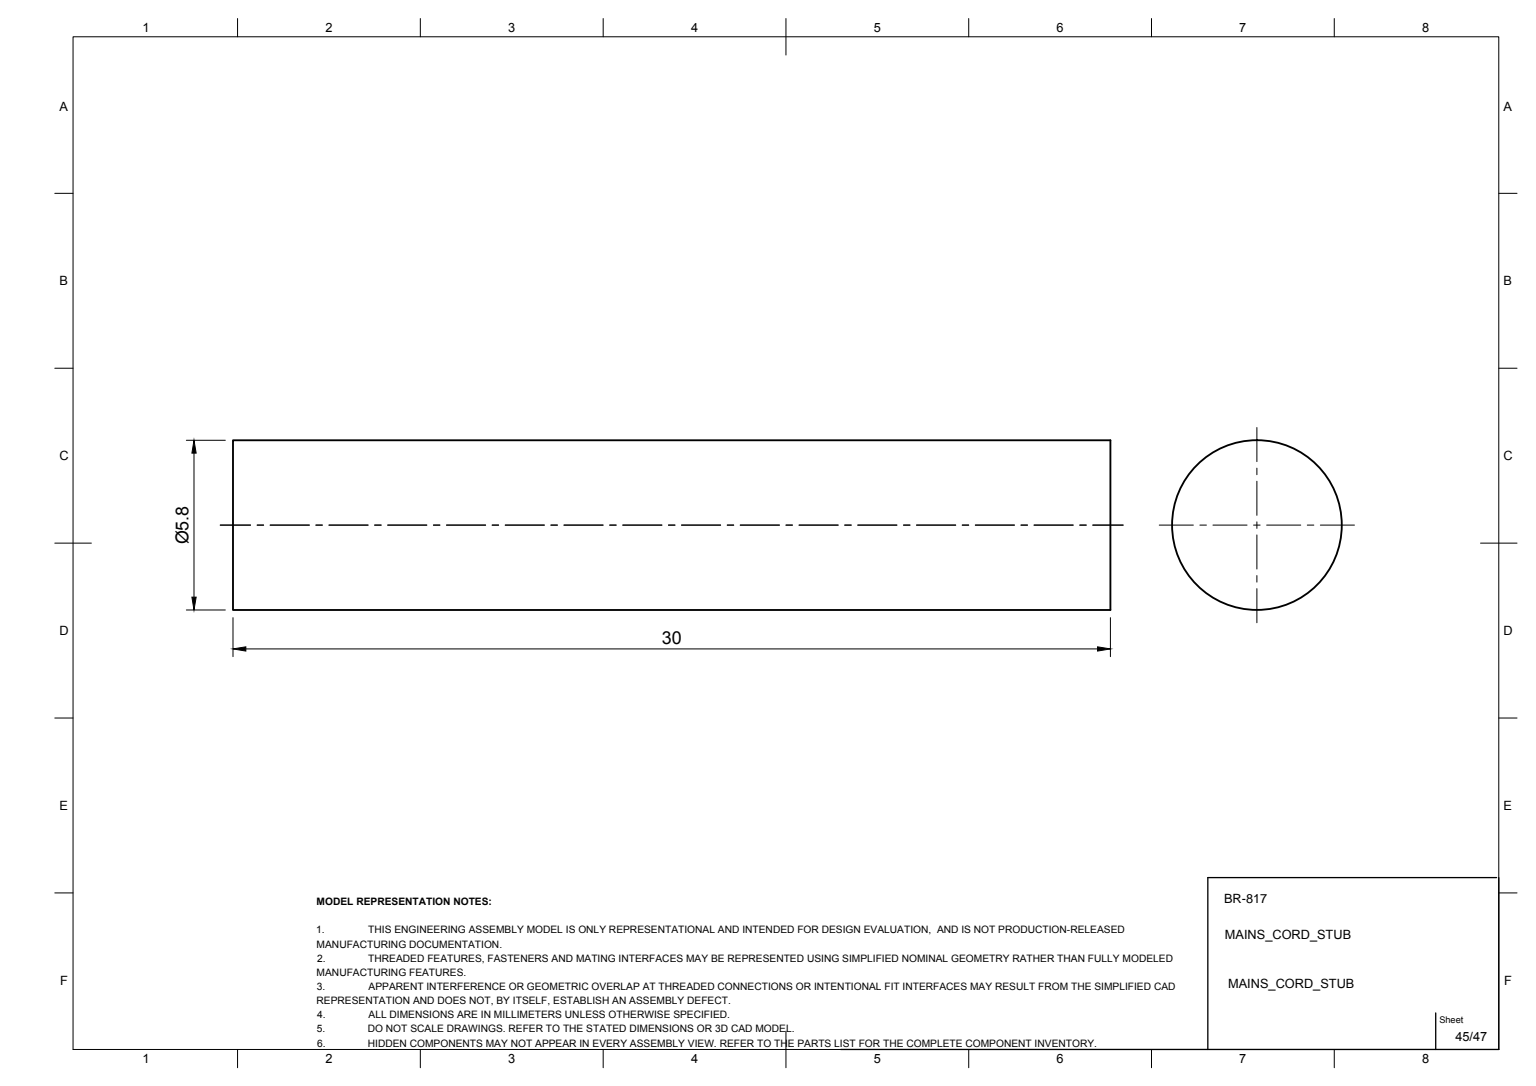
ISO-10303-21;
HEADER;
FILE_DESCRIPTION((''),'2;1');
FILE_NAME('MAINS_CORD_STUB.step','2026-10-01T22:07:29-07:00',(''),(''),'','','');
FILE_SCHEMA (('AUTOMOTIVE_DESIGN { 1 0 10303 214 3 1 1 }'));
ENDSEC;
DATA;
#10=MECHANICAL_DESIGN_GEOMETRIC_PRESENTATION_REPRESENTATION('',(#582),#15484);
#505=SHAPE_REPRESENTATION_RELATIONSHIP('SRR','None',#15656,#540) ;
#540=ADVANCED_BREP_SHAPE_REPRESENTATION('',(#623),#15480) ;
#582=STYLED_ITEM('',(#15843),#623) ;
#623=MANIFOLD_SOLID_BREP('MAINS_CORD_STUB',#8293) ;
#805=CYLINDRICAL_SURFACE('',#9880,0.29) ;
#1355=CIRCLE('',#9881,0.29) ;
#1356=CIRCLE('',#9882,0.29) ;
#1852=FACE_OUTER_BOUND('',#2425,.T.) ;
#1853=FACE_OUTER_BOUND('',#2426,.T.) ;
#1854=FACE_OUTER_BOUND('',#2427,.T.) ;
#2425=EDGE_LOOP('',(#7507,#7508,#7509,#7510)) ;
#2426=EDGE_LOOP('',(#7511)) ;
#2427=EDGE_LOOP('',(#7512)) ;
#2909=LINE('',#15343,#3383) ;
#3383=VECTOR('',#12794,0.29) ;
#4131=VERTEX_POINT('',#15340) ;
#4132=VERTEX_POINT('',#15342) ;
#5258=EDGE_CURVE('',#4131,#4131,#1355,.T.) ;
#5259=EDGE_CURVE('',#4131,#4132,#2909,.T.) ;
#5260=EDGE_CURVE('',#4132,#4132,#1356,.T.) ;
#7507=ORIENTED_EDGE('',*,*,#5258,.F.) ;
#7508=ORIENTED_EDGE('',*,*,#5259,.T.) ;
#7509=ORIENTED_EDGE('',*,*,#5260,.F.) ;
#7510=ORIENTED_EDGE('',*,*,#5259,.F.) ;
#7511=ORIENTED_EDGE('',*,*,#5260,.T.) ;
#7512=ORIENTED_EDGE('',*,*,#5258,.T.) ;
#7744=PLANE('',#9883) ;
#7745=PLANE('',#9884) ;
#8239=ADVANCED_FACE('',(#1852),#805,.T.) ;
#8240=ADVANCED_FACE('',(#1853),#7744,.T.) ;
#8241=ADVANCED_FACE('',(#1854),#7745,.T.) ;
#8293=CLOSED_SHELL('',(#8239,#8240,#8241)) ;
#9879=AXIS2_PLACEMENT_3D('',#15338,#12788,#12789) ;
#9880=AXIS2_PLACEMENT_3D('',#15339,#12790,#12791) ;
#9881=AXIS2_PLACEMENT_3D('',#15341,#12792,#12793) ;
#9882=AXIS2_PLACEMENT_3D('',#15344,#12795,#12796) ;
#9883=AXIS2_PLACEMENT_3D('',#15345,#12797,#12798) ;
#9884=AXIS2_PLACEMENT_3D('',#15346,#12799,#12800) ;
#12788=DIRECTION('axis',(0.,0.,1.)) ;
#12789=DIRECTION('refdir',(1.,0.,0.)) ;
#12790=DIRECTION('center_axis',(1.,0.,0.)) ;
#12791=DIRECTION('ref_axis',(0.,0.,-1.)) ;
#12792=DIRECTION('center_axis',(1.,0.,0.)) ;
#12793=DIRECTION('ref_axis',(0.,0.,-1.)) ;
#12794=DIRECTION('',(-1.,0.,0.)) ;
#12795=DIRECTION('center_axis',(-1.,0.,0.)) ;
#12796=DIRECTION('ref_axis',(0.,0.,-1.)) ;
#12797=DIRECTION('center_axis',(-1.,0.,0.)) ;
#12798=DIRECTION('ref_axis',(0.,0.,1.)) ;
#12799=DIRECTION('center_axis',(1.,0.,0.)) ;
#12800=DIRECTION('ref_axis',(0.,0.,-1.)) ;
#15338=CARTESIAN_POINT('',(0.,0.,0.)) ;
#15339=CARTESIAN_POINT('Origin',(2.5,-1.6,-0.4)) ;
#15340=CARTESIAN_POINT('',(4.,-1.6,-0.11)) ;
#15341=CARTESIAN_POINT('Origin',(4.,-1.6,-0.4)) ;
#15342=CARTESIAN_POINT('',(1.,-1.6,-0.11)) ;
#15343=CARTESIAN_POINT('',(2.5,-1.6,-0.11)) ;
#15344=CARTESIAN_POINT('Origin',(1.,-1.6,-0.4)) ;
#15345=CARTESIAN_POINT('Origin',(1.,-1.6,-0.4)) ;
#15346=CARTESIAN_POINT('Origin',(4.,-1.6,-0.4)) ;
#15437=UNCERTAINTY_MEASURE_WITH_UNIT(LENGTH_MEASURE(0.001),#15485,
'DISTANCE_ACCURACY_VALUE',
'Maximum model space distance between geometric entities at asserted c
onnectivities') ;
#15441=UNCERTAINTY_MEASURE_WITH_UNIT(LENGTH_MEASURE(0.001),#15485,
'DISTANCE_ACCURACY_VALUE',
'Maximum model space distance between geometric entities at asserted c
onnectivities') ;
#15480=(
GEOMETRIC_REPRESENTATION_CONTEXT(3)
GLOBAL_UNCERTAINTY_ASSIGNED_CONTEXT((#15437))
GLOBAL_UNIT_ASSIGNED_CONTEXT((#15485,#15487,#15488))
REPRESENTATION_CONTEXT('','3D')
) ;
#15484=(
GEOMETRIC_REPRESENTATION_CONTEXT(3)
GLOBAL_UNCERTAINTY_ASSIGNED_CONTEXT((#15441))
GLOBAL_UNIT_ASSIGNED_CONTEXT((#15485,#15487,#15488))
REPRESENTATION_CONTEXT('','3D')
) ;
#15485=(
LENGTH_UNIT()
NAMED_UNIT(*)
SI_UNIT(.CENTI.,.METRE.)
) ;
#15487=(
NAMED_UNIT(*)
PLANE_ANGLE_UNIT()
SI_UNIT($,.RADIAN.)
) ;
#15488=(
NAMED_UNIT(*)
SI_UNIT($,.STERADIAN.)
SOLID_ANGLE_UNIT()
) ;
#15527=SHAPE_DEFINITION_REPRESENTATION(#15595,#15656) ;
#15595=PRODUCT_DEFINITION_SHAPE('',$,#15699) ;
#15656=SHAPE_REPRESENTATION('',(#9879),#15480) ;
#15660=PRODUCT_DEFINITION_CONTEXT('part definition',#15788,'design') ;
#15699=PRODUCT_DEFINITION('MAINS_CORD_STUB','MAINS_CORD_STUB',#15741,
#15660) ;
#15741=PRODUCT_DEFINITION_FORMATION('',$,#15828) ;
#15788=APPLICATION_CONTEXT(
'Core Data for Automotive Mechanical Design Process') ;
#15789=PRODUCT_CONTEXT('part definition',#15788,'mechanical') ;
#15828=PRODUCT('MAINS_CORD_STUB','MAINS_CORD_STUB',$,(#15789)) ;
#15843=PRESENTATION_STYLE_ASSIGNMENT((#15855)) ;
#15855=SURFACE_STYLE_USAGE(.BOTH.,#15867) ;
#15867=SURFACE_SIDE_STYLE('',(#15879)) ;
#15879=SURFACE_STYLE_FILL_AREA(#15891) ;
#15891=FILL_AREA_STYLE('Rubber - Soft',(#15903)) ;
#15903=FILL_AREA_STYLE_COLOUR('Rubber - Soft',#15915) ;
#15915=COLOUR_RGB('Rubber - Soft', 0.72549020, 0.75294118, 0.79215686) ;
ENDSEC;
END-ISO-10303-21;
